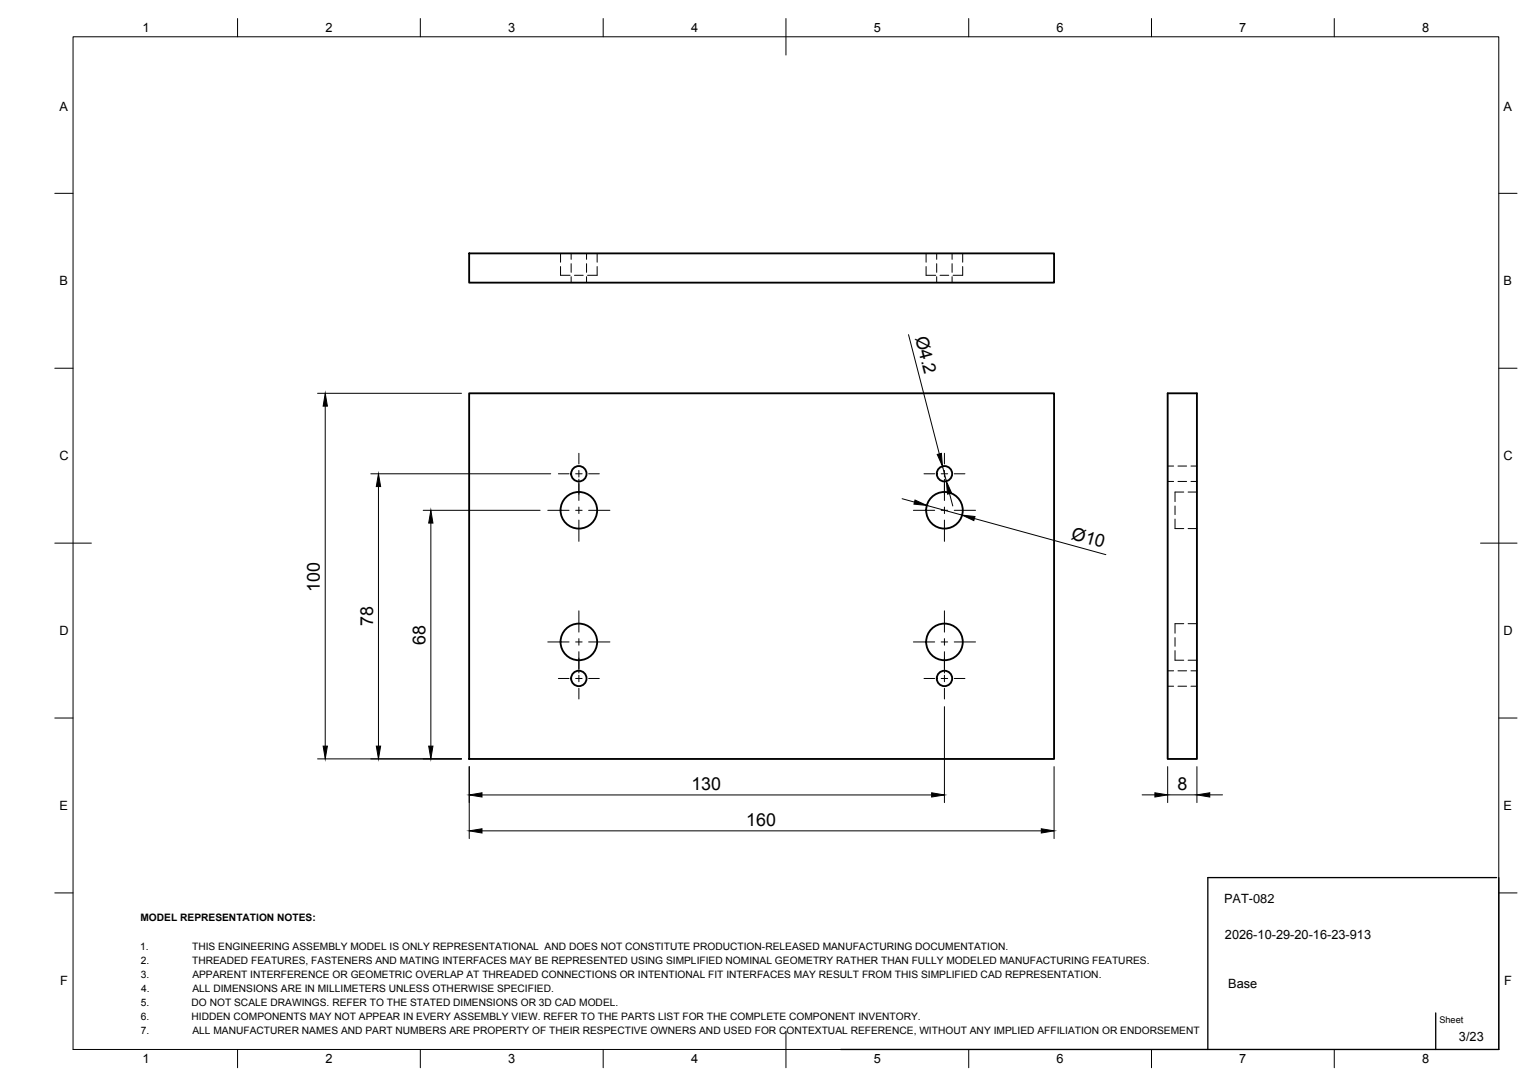
ISO-10303-21;
HEADER;
/* Generated by software containing ST-Developer
 * from STEP Tools, Inc. (www.steptools.com) 
 */

FILE_DESCRIPTION(
/* description */ ('PAT-082'),
/* implementation_level */ '2;1');

FILE_NAME(
/* name */ 'Base.step',
/* time_stamp */ '2026-10-29T20:16:13-07:00',
/* author */ (''),
/* organization */ (''),
/* preprocessor_version */ 'ST-DEVELOPER v20.2',
/* originating_system */ 'Autodesk Translation Framework v15.17.0.0',
/* authorisation */ '');

FILE_SCHEMA (('AUTOMOTIVE_DESIGN { 1 0 10303 214 3 1 1 }'));
ENDSEC;

DATA;
#10=MECHANICAL_DESIGN_GEOMETRIC_PRESENTATION_REPRESENTATION('',(#241),#8266);
#197=SHAPE_REPRESENTATION_RELATIONSHIP('SRR','None',#8359,#219);
#219=ADVANCED_BREP_SHAPE_REPRESENTATION('',(#263),#8243);
#241=STYLED_ITEM('',(#8516),#263);
#263=MANIFOLD_SOLID_BREP('Body1',#4581);
#282=FACE_BOUND('',#859,.T.);
#283=FACE_BOUND('',#860,.T.);
#284=FACE_BOUND('',#861,.T.);
#285=FACE_BOUND('',#862,.T.);
#286=FACE_BOUND('',#863,.T.);
#287=FACE_BOUND('',#864,.T.);
#288=FACE_BOUND('',#865,.T.);
#289=FACE_BOUND('',#866,.T.);
#290=FACE_BOUND('',#868,.T.);
#291=FACE_BOUND('',#869,.T.);
#292=FACE_BOUND('',#870,.T.);
#293=FACE_BOUND('',#871,.T.);
#405=PLANE('',#4854);
#406=PLANE('',#4858);
#407=PLANE('',#4862);
#408=PLANE('',#4866);
#409=PLANE('',#4879);
#410=PLANE('',#4880);
#411=PLANE('',#4881);
#412=PLANE('',#4882);
#413=PLANE('',#4883);
#414=PLANE('',#4884);
#572=FACE_OUTER_BOUND('',#842,.T.);
#573=FACE_OUTER_BOUND('',#843,.T.);
#574=FACE_OUTER_BOUND('',#844,.T.);
#575=FACE_OUTER_BOUND('',#845,.T.);
#576=FACE_OUTER_BOUND('',#846,.T.);
#577=FACE_OUTER_BOUND('',#847,.T.);
#578=FACE_OUTER_BOUND('',#848,.T.);
#579=FACE_OUTER_BOUND('',#849,.T.);
#580=FACE_OUTER_BOUND('',#850,.T.);
#581=FACE_OUTER_BOUND('',#851,.T.);
#582=FACE_OUTER_BOUND('',#852,.T.);
#583=FACE_OUTER_BOUND('',#853,.T.);
#584=FACE_OUTER_BOUND('',#854,.T.);
#585=FACE_OUTER_BOUND('',#855,.T.);
#586=FACE_OUTER_BOUND('',#856,.T.);
#587=FACE_OUTER_BOUND('',#857,.T.);
#588=FACE_OUTER_BOUND('',#858,.T.);
#589=FACE_OUTER_BOUND('',#867,.T.);
#842=EDGE_LOOP('',(#3086,#3087,#3088,#3089));
#843=EDGE_LOOP('',(#3090));
#844=EDGE_LOOP('',(#3091,#3092,#3093,#3094));
#845=EDGE_LOOP('',(#3095));
#846=EDGE_LOOP('',(#3096,#3097,#3098,#3099));
#847=EDGE_LOOP('',(#3100));
#848=EDGE_LOOP('',(#3101,#3102,#3103,#3104));
#849=EDGE_LOOP('',(#3105));
#850=EDGE_LOOP('',(#3106,#3107,#3108,#3109));
#851=EDGE_LOOP('',(#3110,#3111,#3112,#3113));
#852=EDGE_LOOP('',(#3114,#3115,#3116,#3117));
#853=EDGE_LOOP('',(#3118,#3119,#3120,#3121));
#854=EDGE_LOOP('',(#3122,#3123,#3124,#3125));
#855=EDGE_LOOP('',(#3126,#3127,#3128,#3129));
#856=EDGE_LOOP('',(#3130,#3131,#3132,#3133));
#857=EDGE_LOOP('',(#3134,#3135,#3136,#3137));
#858=EDGE_LOOP('',(#3138,#3139,#3140,#3141));
#859=EDGE_LOOP('',(#3142));
#860=EDGE_LOOP('',(#3143));
#861=EDGE_LOOP('',(#3144));
#862=EDGE_LOOP('',(#3145));
#863=EDGE_LOOP('',(#3146));
#864=EDGE_LOOP('',(#3147));
#865=EDGE_LOOP('',(#3148));
#866=EDGE_LOOP('',(#3149));
#867=EDGE_LOOP('',(#3150,#3151,#3152,#3153));
#868=EDGE_LOOP('',(#3154));
#869=EDGE_LOOP('',(#3155));
#870=EDGE_LOOP('',(#3156));
#871=EDGE_LOOP('',(#3157));
#1235=LINE('',#6809,#1590);
#1236=LINE('',#6816,#1591);
#1237=LINE('',#6823,#1592);
#1238=LINE('',#6830,#1593);
#1239=LINE('',#6837,#1594);
#1240=LINE('',#6843,#1595);
#1241=LINE('',#6849,#1596);
#1242=LINE('',#6855,#1597);
#1243=LINE('',#6860,#1598);
#1244=LINE('',#6862,#1599);
#1245=LINE('',#6864,#1600);
#1246=LINE('',#6865,#1601);
#1247=LINE('',#6868,#1602);
#1248=LINE('',#6870,#1603);
#1249=LINE('',#6871,#1604);
#1250=LINE('',#6874,#1605);
#1251=LINE('',#6876,#1606);
#1252=LINE('',#6877,#1607);
#1253=LINE('',#6879,#1608);
#1254=LINE('',#6880,#1609);
#1590=VECTOR('',#5390,0.5);
#1591=VECTOR('',#5399,0.5);
#1592=VECTOR('',#5408,0.5);
#1593=VECTOR('',#5417,0.5);
#1594=VECTOR('',#5426,0.21);
#1595=VECTOR('',#5433,0.21);
#1596=VECTOR('',#5440,0.21);
#1597=VECTOR('',#5447,0.21);
#1598=VECTOR('',#5452,1.);
#1599=VECTOR('',#5453,1.);
#1600=VECTOR('',#5454,1.);
#1601=VECTOR('',#5455,1.);
#1602=VECTOR('',#5458,1.);
#1603=VECTOR('',#5459,1.);
#1604=VECTOR('',#5460,1.);
#1605=VECTOR('',#5463,1.);
#1606=VECTOR('',#5464,1.);
#1607=VECTOR('',#5465,1.);
#1608=VECTOR('',#5468,1.);
#1609=VECTOR('',#5469,1.);
#1945=CIRCLE('',#4852,0.5);
#1946=CIRCLE('',#4853,0.5);
#1947=CIRCLE('',#4856,0.5);
#1948=CIRCLE('',#4857,0.5);
#1949=CIRCLE('',#4860,0.5);
#1950=CIRCLE('',#4861,0.5);
#1951=CIRCLE('',#4864,0.5);
#1952=CIRCLE('',#4865,0.5);
#1953=CIRCLE('',#4868,0.21);
#1954=CIRCLE('',#4869,0.21);
#1955=CIRCLE('',#4871,0.21);
#1956=CIRCLE('',#4872,0.21);
#1957=CIRCLE('',#4874,0.21);
#1958=CIRCLE('',#4875,0.21);
#1959=CIRCLE('',#4877,0.21);
#1960=CIRCLE('',#4878,0.21);
#2145=VERTEX_POINT('',#6806);
#2146=VERTEX_POINT('',#6808);
#2147=VERTEX_POINT('',#6813);
#2148=VERTEX_POINT('',#6815);
#2149=VERTEX_POINT('',#6820);
#2150=VERTEX_POINT('',#6822);
#2151=VERTEX_POINT('',#6827);
#2152=VERTEX_POINT('',#6829);
#2153=VERTEX_POINT('',#6834);
#2154=VERTEX_POINT('',#6836);
#2155=VERTEX_POINT('',#6840);
#2156=VERTEX_POINT('',#6842);
#2157=VERTEX_POINT('',#6846);
#2158=VERTEX_POINT('',#6848);
#2159=VERTEX_POINT('',#6852);
#2160=VERTEX_POINT('',#6854);
#2161=VERTEX_POINT('',#6858);
#2162=VERTEX_POINT('',#6859);
#2163=VERTEX_POINT('',#6861);
#2164=VERTEX_POINT('',#6863);
#2165=VERTEX_POINT('',#6867);
#2166=VERTEX_POINT('',#6869);
#2167=VERTEX_POINT('',#6873);
#2168=VERTEX_POINT('',#6875);
#2519=EDGE_CURVE('',#2145,#2145,#1945,.T.);
#2520=EDGE_CURVE('',#2145,#2146,#1235,.T.);
#2521=EDGE_CURVE('',#2146,#2146,#1946,.T.);
#2522=EDGE_CURVE('',#2147,#2147,#1947,.T.);
#2523=EDGE_CURVE('',#2147,#2148,#1236,.T.);
#2524=EDGE_CURVE('',#2148,#2148,#1948,.T.);
#2525=EDGE_CURVE('',#2149,#2149,#1949,.T.);
#2526=EDGE_CURVE('',#2149,#2150,#1237,.T.);
#2527=EDGE_CURVE('',#2150,#2150,#1950,.T.);
#2528=EDGE_CURVE('',#2151,#2151,#1951,.T.);
#2529=EDGE_CURVE('',#2151,#2152,#1238,.T.);
#2530=EDGE_CURVE('',#2152,#2152,#1952,.T.);
#2531=EDGE_CURVE('',#2153,#2153,#1953,.T.);
#2532=EDGE_CURVE('',#2153,#2154,#1239,.T.);
#2533=EDGE_CURVE('',#2154,#2154,#1954,.T.);
#2534=EDGE_CURVE('',#2155,#2155,#1955,.T.);
#2535=EDGE_CURVE('',#2155,#2156,#1240,.T.);
#2536=EDGE_CURVE('',#2156,#2156,#1956,.T.);
#2537=EDGE_CURVE('',#2157,#2157,#1957,.T.);
#2538=EDGE_CURVE('',#2157,#2158,#1241,.T.);
#2539=EDGE_CURVE('',#2158,#2158,#1958,.T.);
#2540=EDGE_CURVE('',#2159,#2159,#1959,.T.);
#2541=EDGE_CURVE('',#2159,#2160,#1242,.T.);
#2542=EDGE_CURVE('',#2160,#2160,#1960,.T.);
#2543=EDGE_CURVE('',#2161,#2162,#1243,.T.);
#2544=EDGE_CURVE('',#2162,#2163,#1244,.T.);
#2545=EDGE_CURVE('',#2164,#2163,#1245,.T.);
#2546=EDGE_CURVE('',#2161,#2164,#1246,.T.);
#2547=EDGE_CURVE('',#2165,#2161,#1247,.T.);
#2548=EDGE_CURVE('',#2166,#2164,#1248,.T.);
#2549=EDGE_CURVE('',#2165,#2166,#1249,.T.);
#2550=EDGE_CURVE('',#2167,#2165,#1250,.T.);
#2551=EDGE_CURVE('',#2168,#2166,#1251,.T.);
#2552=EDGE_CURVE('',#2167,#2168,#1252,.T.);
#2553=EDGE_CURVE('',#2162,#2167,#1253,.T.);
#2554=EDGE_CURVE('',#2163,#2168,#1254,.T.);
#3086=ORIENTED_EDGE('',*,*,#2519,.F.);
#3087=ORIENTED_EDGE('',*,*,#2520,.T.);
#3088=ORIENTED_EDGE('',*,*,#2521,.F.);
#3089=ORIENTED_EDGE('',*,*,#2520,.F.);
#3090=ORIENTED_EDGE('',*,*,#2519,.T.);
#3091=ORIENTED_EDGE('',*,*,#2522,.F.);
#3092=ORIENTED_EDGE('',*,*,#2523,.T.);
#3093=ORIENTED_EDGE('',*,*,#2524,.F.);
#3094=ORIENTED_EDGE('',*,*,#2523,.F.);
#3095=ORIENTED_EDGE('',*,*,#2522,.T.);
#3096=ORIENTED_EDGE('',*,*,#2525,.F.);
#3097=ORIENTED_EDGE('',*,*,#2526,.T.);
#3098=ORIENTED_EDGE('',*,*,#2527,.F.);
#3099=ORIENTED_EDGE('',*,*,#2526,.F.);
#3100=ORIENTED_EDGE('',*,*,#2525,.T.);
#3101=ORIENTED_EDGE('',*,*,#2528,.F.);
#3102=ORIENTED_EDGE('',*,*,#2529,.T.);
#3103=ORIENTED_EDGE('',*,*,#2530,.F.);
#3104=ORIENTED_EDGE('',*,*,#2529,.F.);
#3105=ORIENTED_EDGE('',*,*,#2528,.T.);
#3106=ORIENTED_EDGE('',*,*,#2531,.F.);
#3107=ORIENTED_EDGE('',*,*,#2532,.T.);
#3108=ORIENTED_EDGE('',*,*,#2533,.F.);
#3109=ORIENTED_EDGE('',*,*,#2532,.F.);
#3110=ORIENTED_EDGE('',*,*,#2534,.F.);
#3111=ORIENTED_EDGE('',*,*,#2535,.T.);
#3112=ORIENTED_EDGE('',*,*,#2536,.F.);
#3113=ORIENTED_EDGE('',*,*,#2535,.F.);
#3114=ORIENTED_EDGE('',*,*,#2537,.F.);
#3115=ORIENTED_EDGE('',*,*,#2538,.T.);
#3116=ORIENTED_EDGE('',*,*,#2539,.F.);
#3117=ORIENTED_EDGE('',*,*,#2538,.F.);
#3118=ORIENTED_EDGE('',*,*,#2540,.F.);
#3119=ORIENTED_EDGE('',*,*,#2541,.T.);
#3120=ORIENTED_EDGE('',*,*,#2542,.F.);
#3121=ORIENTED_EDGE('',*,*,#2541,.F.);
#3122=ORIENTED_EDGE('',*,*,#2543,.T.);
#3123=ORIENTED_EDGE('',*,*,#2544,.T.);
#3124=ORIENTED_EDGE('',*,*,#2545,.F.);
#3125=ORIENTED_EDGE('',*,*,#2546,.F.);
#3126=ORIENTED_EDGE('',*,*,#2547,.T.);
#3127=ORIENTED_EDGE('',*,*,#2546,.T.);
#3128=ORIENTED_EDGE('',*,*,#2548,.F.);
#3129=ORIENTED_EDGE('',*,*,#2549,.F.);
#3130=ORIENTED_EDGE('',*,*,#2550,.T.);
#3131=ORIENTED_EDGE('',*,*,#2549,.T.);
#3132=ORIENTED_EDGE('',*,*,#2551,.F.);
#3133=ORIENTED_EDGE('',*,*,#2552,.F.);
#3134=ORIENTED_EDGE('',*,*,#2553,.T.);
#3135=ORIENTED_EDGE('',*,*,#2552,.T.);
#3136=ORIENTED_EDGE('',*,*,#2554,.F.);
#3137=ORIENTED_EDGE('',*,*,#2544,.F.);
#3138=ORIENTED_EDGE('',*,*,#2554,.T.);
#3139=ORIENTED_EDGE('',*,*,#2551,.T.);
#3140=ORIENTED_EDGE('',*,*,#2548,.T.);
#3141=ORIENTED_EDGE('',*,*,#2545,.T.);
#3142=ORIENTED_EDGE('',*,*,#2542,.T.);
#3143=ORIENTED_EDGE('',*,*,#2539,.T.);
#3144=ORIENTED_EDGE('',*,*,#2536,.T.);
#3145=ORIENTED_EDGE('',*,*,#2533,.T.);
#3146=ORIENTED_EDGE('',*,*,#2530,.T.);
#3147=ORIENTED_EDGE('',*,*,#2527,.T.);
#3148=ORIENTED_EDGE('',*,*,#2524,.T.);
#3149=ORIENTED_EDGE('',*,*,#2521,.T.);
#3150=ORIENTED_EDGE('',*,*,#2553,.F.);
#3151=ORIENTED_EDGE('',*,*,#2543,.F.);
#3152=ORIENTED_EDGE('',*,*,#2547,.F.);
#3153=ORIENTED_EDGE('',*,*,#2550,.F.);
#3154=ORIENTED_EDGE('',*,*,#2531,.T.);
#3155=ORIENTED_EDGE('',*,*,#2534,.T.);
#3156=ORIENTED_EDGE('',*,*,#2537,.T.);
#3157=ORIENTED_EDGE('',*,*,#2540,.T.);
#4220=CYLINDRICAL_SURFACE('',#4851,0.5);
#4221=CYLINDRICAL_SURFACE('',#4855,0.5);
#4222=CYLINDRICAL_SURFACE('',#4859,0.5);
#4223=CYLINDRICAL_SURFACE('',#4863,0.5);
#4224=CYLINDRICAL_SURFACE('',#4867,0.21);
#4225=CYLINDRICAL_SURFACE('',#4870,0.21);
#4226=CYLINDRICAL_SURFACE('',#4873,0.21);
#4227=CYLINDRICAL_SURFACE('',#4876,0.21);
#4311=ADVANCED_FACE('',(#572),#4220,.F.);
#4312=ADVANCED_FACE('',(#573),#405,.T.);
#4313=ADVANCED_FACE('',(#574),#4221,.F.);
#4314=ADVANCED_FACE('',(#575),#406,.T.);
#4315=ADVANCED_FACE('',(#576),#4222,.F.);
#4316=ADVANCED_FACE('',(#577),#407,.T.);
#4317=ADVANCED_FACE('',(#578),#4223,.F.);
#4318=ADVANCED_FACE('',(#579),#408,.T.);
#4319=ADVANCED_FACE('',(#580),#4224,.F.);
#4320=ADVANCED_FACE('',(#581),#4225,.F.);
#4321=ADVANCED_FACE('',(#582),#4226,.F.);
#4322=ADVANCED_FACE('',(#583),#4227,.F.);
#4323=ADVANCED_FACE('',(#584),#409,.T.);
#4324=ADVANCED_FACE('',(#585),#410,.T.);
#4325=ADVANCED_FACE('',(#586),#411,.T.);
#4326=ADVANCED_FACE('',(#587),#412,.T.);
#4327=ADVANCED_FACE('',(#588,#282,#283,#284,#285,#286,#287,#288,#289),#413,
 .T.);
#4328=ADVANCED_FACE('',(#589,#290,#291,#292,#293),#414,.F.);
#4581=CLOSED_SHELL('',(#4311,#4312,#4313,#4314,#4315,#4316,#4317,#4318,
#4319,#4320,#4321,#4322,#4323,#4324,#4325,#4326,#4327,#4328));
#4850=AXIS2_PLACEMENT_3D('',#6804,#5384,#5385);
#4851=AXIS2_PLACEMENT_3D('',#6805,#5386,#5387);
#4852=AXIS2_PLACEMENT_3D('',#6807,#5388,#5389);
#4853=AXIS2_PLACEMENT_3D('',#6810,#5391,#5392);
#4854=AXIS2_PLACEMENT_3D('',#6811,#5393,#5394);
#4855=AXIS2_PLACEMENT_3D('',#6812,#5395,#5396);
#4856=AXIS2_PLACEMENT_3D('',#6814,#5397,#5398);
#4857=AXIS2_PLACEMENT_3D('',#6817,#5400,#5401);
#4858=AXIS2_PLACEMENT_3D('',#6818,#5402,#5403);
#4859=AXIS2_PLACEMENT_3D('',#6819,#5404,#5405);
#4860=AXIS2_PLACEMENT_3D('',#6821,#5406,#5407);
#4861=AXIS2_PLACEMENT_3D('',#6824,#5409,#5410);
#4862=AXIS2_PLACEMENT_3D('',#6825,#5411,#5412);
#4863=AXIS2_PLACEMENT_3D('',#6826,#5413,#5414);
#4864=AXIS2_PLACEMENT_3D('',#6828,#5415,#5416);
#4865=AXIS2_PLACEMENT_3D('',#6831,#5418,#5419);
#4866=AXIS2_PLACEMENT_3D('',#6832,#5420,#5421);
#4867=AXIS2_PLACEMENT_3D('',#6833,#5422,#5423);
#4868=AXIS2_PLACEMENT_3D('',#6835,#5424,#5425);
#4869=AXIS2_PLACEMENT_3D('',#6838,#5427,#5428);
#4870=AXIS2_PLACEMENT_3D('',#6839,#5429,#5430);
#4871=AXIS2_PLACEMENT_3D('',#6841,#5431,#5432);
#4872=AXIS2_PLACEMENT_3D('',#6844,#5434,#5435);
#4873=AXIS2_PLACEMENT_3D('',#6845,#5436,#5437);
#4874=AXIS2_PLACEMENT_3D('',#6847,#5438,#5439);
#4875=AXIS2_PLACEMENT_3D('',#6850,#5441,#5442);
#4876=AXIS2_PLACEMENT_3D('',#6851,#5443,#5444);
#4877=AXIS2_PLACEMENT_3D('',#6853,#5445,#5446);
#4878=AXIS2_PLACEMENT_3D('',#6856,#5448,#5449);
#4879=AXIS2_PLACEMENT_3D('',#6857,#5450,#5451);
#4880=AXIS2_PLACEMENT_3D('',#6866,#5456,#5457);
#4881=AXIS2_PLACEMENT_3D('',#6872,#5461,#5462);
#4882=AXIS2_PLACEMENT_3D('',#6878,#5466,#5467);
#4883=AXIS2_PLACEMENT_3D('',#6881,#5470,#5471);
#4884=AXIS2_PLACEMENT_3D('',#6882,#5472,#5473);
#5384=DIRECTION('axis',(0.,0.,1.));
#5385=DIRECTION('refdir',(1.,0.,0.));
#5386=DIRECTION('center_axis',(0.,0.,1.));
#5387=DIRECTION('ref_axis',(1.,0.,0.));
#5388=DIRECTION('center_axis',(0.,0.,1.));
#5389=DIRECTION('ref_axis',(1.,0.,0.));
#5390=DIRECTION('',(0.,0.,1.));
#5391=DIRECTION('center_axis',(0.,0.,-1.));
#5392=DIRECTION('ref_axis',(1.,0.,0.));
#5393=DIRECTION('center_axis',(0.,0.,1.));
#5394=DIRECTION('ref_axis',(1.,0.,0.));
#5395=DIRECTION('center_axis',(0.,0.,1.));
#5396=DIRECTION('ref_axis',(1.,0.,0.));
#5397=DIRECTION('center_axis',(0.,0.,1.));
#5398=DIRECTION('ref_axis',(1.,0.,0.));
#5399=DIRECTION('',(0.,0.,1.));
#5400=DIRECTION('center_axis',(0.,0.,-1.));
#5401=DIRECTION('ref_axis',(1.,0.,0.));
#5402=DIRECTION('center_axis',(0.,0.,1.));
#5403=DIRECTION('ref_axis',(1.,0.,0.));
#5404=DIRECTION('center_axis',(0.,0.,1.));
#5405=DIRECTION('ref_axis',(1.,0.,0.));
#5406=DIRECTION('center_axis',(0.,0.,1.));
#5407=DIRECTION('ref_axis',(1.,0.,0.));
#5408=DIRECTION('',(0.,0.,1.));
#5409=DIRECTION('center_axis',(0.,0.,-1.));
#5410=DIRECTION('ref_axis',(1.,0.,0.));
#5411=DIRECTION('center_axis',(0.,0.,1.));
#5412=DIRECTION('ref_axis',(1.,0.,0.));
#5413=DIRECTION('center_axis',(0.,0.,1.));
#5414=DIRECTION('ref_axis',(1.,0.,0.));
#5415=DIRECTION('center_axis',(0.,0.,1.));
#5416=DIRECTION('ref_axis',(1.,0.,0.));
#5417=DIRECTION('',(0.,0.,1.));
#5418=DIRECTION('center_axis',(0.,0.,-1.));
#5419=DIRECTION('ref_axis',(1.,0.,0.));
#5420=DIRECTION('center_axis',(0.,0.,1.));
#5421=DIRECTION('ref_axis',(1.,0.,0.));
#5422=DIRECTION('center_axis',(0.,0.,1.));
#5423=DIRECTION('ref_axis',(1.,0.,0.));
#5424=DIRECTION('center_axis',(0.,0.,1.));
#5425=DIRECTION('ref_axis',(1.,0.,0.));
#5426=DIRECTION('',(0.,0.,1.));
#5427=DIRECTION('center_axis',(0.,0.,-1.));
#5428=DIRECTION('ref_axis',(1.,0.,0.));
#5429=DIRECTION('center_axis',(0.,0.,1.));
#5430=DIRECTION('ref_axis',(1.,0.,0.));
#5431=DIRECTION('center_axis',(0.,0.,1.));
#5432=DIRECTION('ref_axis',(1.,0.,0.));
#5433=DIRECTION('',(0.,0.,1.));
#5434=DIRECTION('center_axis',(0.,0.,-1.));
#5435=DIRECTION('ref_axis',(1.,0.,0.));
#5436=DIRECTION('center_axis',(0.,0.,1.));
#5437=DIRECTION('ref_axis',(1.,0.,0.));
#5438=DIRECTION('center_axis',(0.,0.,1.));
#5439=DIRECTION('ref_axis',(1.,0.,0.));
#5440=DIRECTION('',(0.,0.,1.));
#5441=DIRECTION('center_axis',(0.,0.,-1.));
#5442=DIRECTION('ref_axis',(1.,0.,0.));
#5443=DIRECTION('center_axis',(0.,0.,1.));
#5444=DIRECTION('ref_axis',(1.,0.,0.));
#5445=DIRECTION('center_axis',(0.,0.,1.));
#5446=DIRECTION('ref_axis',(1.,0.,0.));
#5447=DIRECTION('',(0.,0.,1.));
#5448=DIRECTION('center_axis',(0.,0.,-1.));
#5449=DIRECTION('ref_axis',(1.,0.,0.));
#5450=DIRECTION('center_axis',(0.,1.,0.));
#5451=DIRECTION('ref_axis',(-1.,0.,0.));
#5452=DIRECTION('',(-1.,0.,0.));
#5453=DIRECTION('',(0.,0.,1.));
#5454=DIRECTION('',(-1.,0.,0.));
#5455=DIRECTION('',(0.,0.,1.));
#5456=DIRECTION('center_axis',(1.,0.,0.));
#5457=DIRECTION('ref_axis',(0.,1.,0.));
#5458=DIRECTION('',(0.,1.,0.));
#5459=DIRECTION('',(0.,1.,0.));
#5460=DIRECTION('',(0.,0.,1.));
#5461=DIRECTION('center_axis',(0.,-1.,0.));
#5462=DIRECTION('ref_axis',(1.,0.,0.));
#5463=DIRECTION('',(1.,0.,0.));
#5464=DIRECTION('',(1.,0.,0.));
#5465=DIRECTION('',(0.,0.,1.));
#5466=DIRECTION('center_axis',(-1.,0.,0.));
#5467=DIRECTION('ref_axis',(0.,-1.,0.));
#5468=DIRECTION('',(0.,-1.,0.));
#5469=DIRECTION('',(0.,-1.,0.));
#5470=DIRECTION('center_axis',(0.,0.,1.));
#5471=DIRECTION('ref_axis',(1.,0.,0.));
#5472=DIRECTION('center_axis',(0.,0.,1.));
#5473=DIRECTION('ref_axis',(1.,0.,0.));
#6804=CARTESIAN_POINT('',(0.,0.,0.));
#6805=CARTESIAN_POINT('Origin',(5.,-1.8,-0.2));
#6806=CARTESIAN_POINT('',(4.5,-1.8,-0.2));
#6807=CARTESIAN_POINT('Origin',(5.,-1.8,-0.2));
#6808=CARTESIAN_POINT('',(4.5,-1.8,0.4));
#6809=CARTESIAN_POINT('',(4.5,-1.8,-0.2));
#6810=CARTESIAN_POINT('Origin',(5.,-1.8,0.4));
#6811=CARTESIAN_POINT('Origin',(5.,-1.8,-0.2));
#6812=CARTESIAN_POINT('Origin',(-5.,1.8,-0.2));
#6813=CARTESIAN_POINT('',(-5.5,1.8,-0.2));
#6814=CARTESIAN_POINT('Origin',(-5.,1.8,-0.2));
#6815=CARTESIAN_POINT('',(-5.5,1.8,0.4));
#6816=CARTESIAN_POINT('',(-5.5,1.8,-0.2));
#6817=CARTESIAN_POINT('Origin',(-5.,1.8,0.4));
#6818=CARTESIAN_POINT('Origin',(-5.,1.8,-0.2));
#6819=CARTESIAN_POINT('Origin',(-5.,-1.8,-0.2));
#6820=CARTESIAN_POINT('',(-5.5,-1.8,-0.2));
#6821=CARTESIAN_POINT('Origin',(-5.,-1.8,-0.2));
#6822=CARTESIAN_POINT('',(-5.5,-1.8,0.4));
#6823=CARTESIAN_POINT('',(-5.5,-1.8,-0.2));
#6824=CARTESIAN_POINT('Origin',(-5.,-1.8,0.4));
#6825=CARTESIAN_POINT('Origin',(-5.,-1.8,-0.2));
#6826=CARTESIAN_POINT('Origin',(5.,1.8,-0.2));
#6827=CARTESIAN_POINT('',(4.5,1.8,-0.2));
#6828=CARTESIAN_POINT('Origin',(5.,1.8,-0.2));
#6829=CARTESIAN_POINT('',(4.5,1.8,0.4));
#6830=CARTESIAN_POINT('',(4.5,1.8,-0.2));
#6831=CARTESIAN_POINT('Origin',(5.,1.8,0.4));
#6832=CARTESIAN_POINT('Origin',(5.,1.8,-0.2));
#6833=CARTESIAN_POINT('Origin',(5.,-2.8,-0.5));
#6834=CARTESIAN_POINT('',(4.79,-2.8,-0.4));
#6835=CARTESIAN_POINT('Origin',(5.,-2.8,-0.4));
#6836=CARTESIAN_POINT('',(4.79,-2.8,0.4));
#6837=CARTESIAN_POINT('',(4.79,-2.8,-0.5));
#6838=CARTESIAN_POINT('Origin',(5.,-2.8,0.4));
#6839=CARTESIAN_POINT('Origin',(-5.,2.8,-0.5));
#6840=CARTESIAN_POINT('',(-5.21,2.8,-0.4));
#6841=CARTESIAN_POINT('Origin',(-5.,2.8,-0.4));
#6842=CARTESIAN_POINT('',(-5.21,2.8,0.4));
#6843=CARTESIAN_POINT('',(-5.21,2.8,-0.5));
#6844=CARTESIAN_POINT('Origin',(-5.,2.8,0.4));
#6845=CARTESIAN_POINT('Origin',(-5.,-2.8,-0.5));
#6846=CARTESIAN_POINT('',(-5.21,-2.8,-0.4));
#6847=CARTESIAN_POINT('Origin',(-5.,-2.8,-0.4));
#6848=CARTESIAN_POINT('',(-5.21,-2.8,0.4));
#6849=CARTESIAN_POINT('',(-5.21,-2.8,-0.5));
#6850=CARTESIAN_POINT('Origin',(-5.,-2.8,0.4));
#6851=CARTESIAN_POINT('Origin',(5.,2.8,-0.5));
#6852=CARTESIAN_POINT('',(4.79,2.8,-0.4));
#6853=CARTESIAN_POINT('Origin',(5.,2.8,-0.4));
#6854=CARTESIAN_POINT('',(4.79,2.8,0.4));
#6855=CARTESIAN_POINT('',(4.79,2.8,-0.5));
#6856=CARTESIAN_POINT('Origin',(5.,2.8,0.4));
#6857=CARTESIAN_POINT('Origin',(8.,5.,-0.4));
#6858=CARTESIAN_POINT('',(8.,5.,-0.4));
#6859=CARTESIAN_POINT('',(-8.,5.,-0.4));
#6860=CARTESIAN_POINT('',(8.,5.,-0.4));
#6861=CARTESIAN_POINT('',(-8.,5.,0.4));
#6862=CARTESIAN_POINT('',(-8.,5.,-0.4));
#6863=CARTESIAN_POINT('',(8.,5.,0.4));
#6864=CARTESIAN_POINT('',(8.,5.,0.4));
#6865=CARTESIAN_POINT('',(8.,5.,-0.4));
#6866=CARTESIAN_POINT('Origin',(8.,-5.,-0.4));
#6867=CARTESIAN_POINT('',(8.,-5.,-0.4));
#6868=CARTESIAN_POINT('',(8.,-5.,-0.4));
#6869=CARTESIAN_POINT('',(8.,-5.,0.4));
#6870=CARTESIAN_POINT('',(8.,-5.,0.4));
#6871=CARTESIAN_POINT('',(8.,-5.,-0.4));
#6872=CARTESIAN_POINT('Origin',(-8.,-5.,-0.4));
#6873=CARTESIAN_POINT('',(-8.,-5.,-0.4));
#6874=CARTESIAN_POINT('',(-8.,-5.,-0.4));
#6875=CARTESIAN_POINT('',(-8.,-5.,0.4));
#6876=CARTESIAN_POINT('',(-8.,-5.,0.4));
#6877=CARTESIAN_POINT('',(-8.,-5.,-0.4));
#6878=CARTESIAN_POINT('Origin',(-8.,5.,-0.4));
#6879=CARTESIAN_POINT('',(-8.,5.,-0.4));
#6880=CARTESIAN_POINT('',(-8.,5.,0.4));
#6881=CARTESIAN_POINT('Origin',(0.,0.,0.4));
#6882=CARTESIAN_POINT('Origin',(0.,0.,-0.4));
#8218=UNCERTAINTY_MEASURE_WITH_UNIT(LENGTH_MEASURE(0.001),#8267,
'DISTANCE_ACCURACY_VALUE',
'Maximum model space distance between geometric entities at asserted c
onnectivities');
#8241=UNCERTAINTY_MEASURE_WITH_UNIT(LENGTH_MEASURE(0.001),#8267,
'DISTANCE_ACCURACY_VALUE',
'Maximum model space distance between geometric entities at asserted c
onnectivities');
#8243=(
GEOMETRIC_REPRESENTATION_CONTEXT(3)
GLOBAL_UNCERTAINTY_ASSIGNED_CONTEXT((#8218))
GLOBAL_UNIT_ASSIGNED_CONTEXT((#8267,#8269,#8270))
REPRESENTATION_CONTEXT('','3D')
);
#8266=(
GEOMETRIC_REPRESENTATION_CONTEXT(3)
GLOBAL_UNCERTAINTY_ASSIGNED_CONTEXT((#8241))
GLOBAL_UNIT_ASSIGNED_CONTEXT((#8267,#8269,#8270))
REPRESENTATION_CONTEXT('','3D')
);
#8267=(
LENGTH_UNIT()
NAMED_UNIT(*)
SI_UNIT(.CENTI.,.METRE.)
);
#8269=(
NAMED_UNIT(*)
PLANE_ANGLE_UNIT()
SI_UNIT($,.RADIAN.)
);
#8270=(
NAMED_UNIT(*)
SI_UNIT($,.STERADIAN.)
SOLID_ANGLE_UNIT()
);
#8272=SHAPE_DEFINITION_REPRESENTATION(#8296,#8359);
#8296=PRODUCT_DEFINITION_SHAPE('',$,#8384);
#8359=SHAPE_REPRESENTATION('',(#4850),#8243);
#8382=PRODUCT_DEFINITION_CONTEXT('part definition',#8456,'design');
#8384=PRODUCT_DEFINITION('Base','Base',#8408,#8382);
#8408=PRODUCT_DEFINITION_FORMATION('',$,#8459);
#8456=APPLICATION_CONTEXT(
'Core Data for Automotive Mechanical Design Process');
#8457=PRODUCT_CONTEXT('part definition',#8456,'mechanical');
#8459=PRODUCT('Base','Base','Base',(#8457));
#8510=COLOUR_RGB('Dark Blue',0.08,0.2,0.34);
#8511=FILL_AREA_STYLE_COLOUR('',#8510);
#8512=FILL_AREA_STYLE('',(#8511));
#8513=SURFACE_STYLE_FILL_AREA(#8512);
#8514=SURFACE_SIDE_STYLE('',(#8513));
#8515=SURFACE_STYLE_USAGE(.BOTH.,#8514);
#8516=PRESENTATION_STYLE_ASSIGNMENT((#8515));
ENDSEC;
END-ISO-10303-21;
